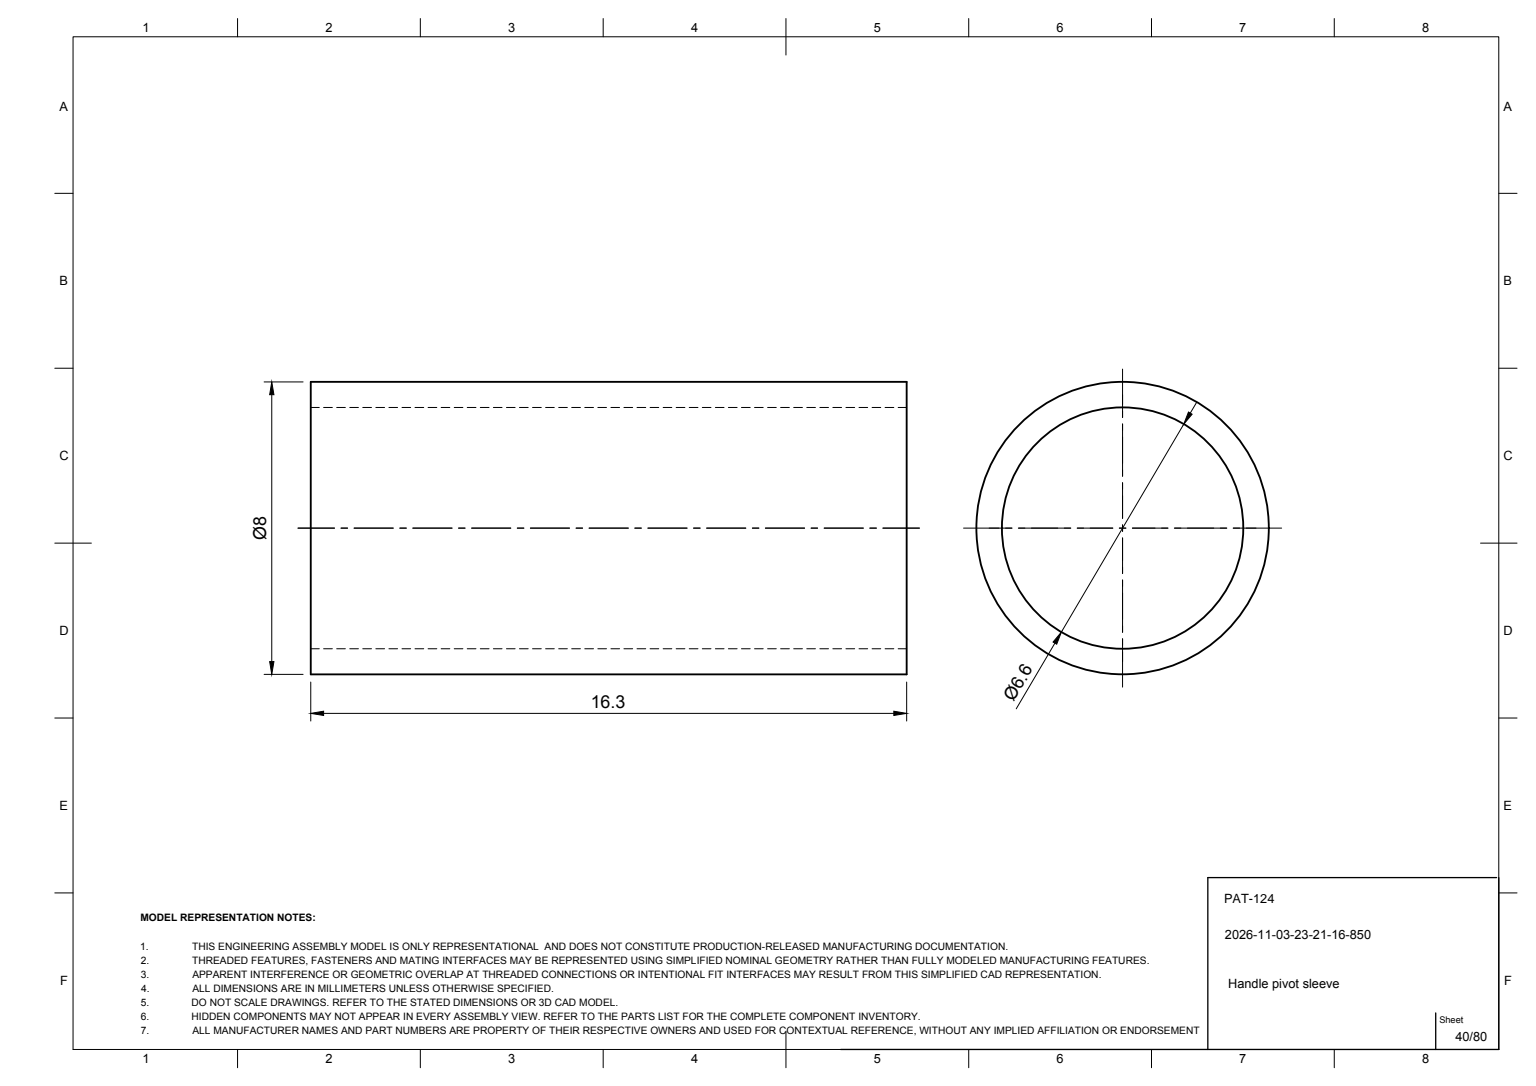
ISO-10303-21;
HEADER;
/* Generated by software containing ST-Developer
 * from STEP Tools, Inc. (www.steptools.com) 
 */

FILE_DESCRIPTION(
/* description */ ('XY cross-slide table'),
/* implementation_level */ '2;1');

FILE_NAME(
/* name */ 'Handle pivot sleeve.step',
/* time_stamp */ '2026-10-28T03:22:46-07:00',
/* author */ (''),
/* organization */ (''),
/* preprocessor_version */ 'ST-DEVELOPER v20.2',
/* originating_system */ 'Autodesk Translation Framework v15.17.0.0',
/* authorisation */ '');

FILE_SCHEMA (('AUTOMOTIVE_DESIGN { 1 0 10303 214 3 1 1 }'));
ENDSEC;

DATA;
#10=MECHANICAL_DESIGN_GEOMETRIC_PRESENTATION_REPRESENTATION('',(#1721),#62984);
#1540=SHAPE_REPRESENTATION_RELATIONSHIP('SRR','None',#63393,#1623);
#1623=ADVANCED_BREP_SHAPE_REPRESENTATION('',(#1831),#62930);
#1721=STYLED_ITEM('',(#63905),#1831);
#1831=MANIFOLD_SOLID_BREP('Body1',#23018);
#2077=FACE_BOUND('',#4968,.T.);
#2078=FACE_BOUND('',#4970,.T.);
#2541=PLANE('',#25079);
#2542=PLANE('',#25080);
#3461=FACE_OUTER_BOUND('',#4965,.T.);
#3462=FACE_OUTER_BOUND('',#4966,.T.);
#3463=FACE_OUTER_BOUND('',#4967,.T.);
#3464=FACE_OUTER_BOUND('',#4969,.T.);
#4965=EDGE_LOOP('',(#17732,#17733,#17734,#17735));
#4966=EDGE_LOOP('',(#17736,#17737,#17738,#17739));
#4967=EDGE_LOOP('',(#17740));
#4968=EDGE_LOOP('',(#17741));
#4969=EDGE_LOOP('',(#17742));
#4970=EDGE_LOOP('',(#17743));
#6569=LINE('',#47517,#8056);
#6570=LINE('',#47523,#8057);
#8056=VECTOR('',#29274,0.33);
#8057=VECTOR('',#29281,0.4);
#9287=CIRCLE('',#25074,0.33);
#9288=CIRCLE('',#25075,0.33);
#9289=CIRCLE('',#25077,0.4);
#9290=CIRCLE('',#25078,0.4);
#10727=VERTEX_POINT('',#47514);
#10728=VERTEX_POINT('',#47516);
#10729=VERTEX_POINT('',#47520);
#10730=VERTEX_POINT('',#47522);
#13250=EDGE_CURVE('',#10727,#10727,#9287,.T.);
#13251=EDGE_CURVE('',#10727,#10728,#6569,.T.);
#13252=EDGE_CURVE('',#10728,#10728,#9288,.T.);
#13253=EDGE_CURVE('',#10729,#10729,#9289,.T.);
#13254=EDGE_CURVE('',#10729,#10730,#6570,.T.);
#13255=EDGE_CURVE('',#10730,#10730,#9290,.T.);
#17732=ORIENTED_EDGE('',*,*,#13250,.F.);
#17733=ORIENTED_EDGE('',*,*,#13251,.T.);
#17734=ORIENTED_EDGE('',*,*,#13252,.T.);
#17735=ORIENTED_EDGE('',*,*,#13251,.F.);
#17736=ORIENTED_EDGE('',*,*,#13253,.F.);
#17737=ORIENTED_EDGE('',*,*,#13254,.T.);
#17738=ORIENTED_EDGE('',*,*,#13255,.T.);
#17739=ORIENTED_EDGE('',*,*,#13254,.F.);
#17740=ORIENTED_EDGE('',*,*,#13253,.T.);
#17741=ORIENTED_EDGE('',*,*,#13250,.T.);
#17742=ORIENTED_EDGE('',*,*,#13255,.F.);
#17743=ORIENTED_EDGE('',*,*,#13252,.F.);
#21329=CYLINDRICAL_SURFACE('',#25073,0.33);
#21330=CYLINDRICAL_SURFACE('',#25076,0.4);
#22242=ADVANCED_FACE('',(#3461),#21329,.F.);
#22243=ADVANCED_FACE('',(#3462),#21330,.T.);
#22244=ADVANCED_FACE('',(#3463,#2077),#2541,.T.);
#22245=ADVANCED_FACE('',(#3464,#2078),#2542,.F.);
#23018=CLOSED_SHELL('',(#22242,#22243,#22244,#22245));
#25072=AXIS2_PLACEMENT_3D('',#47512,#29268,#29269);
#25073=AXIS2_PLACEMENT_3D('',#47513,#29270,#29271);
#25074=AXIS2_PLACEMENT_3D('',#47515,#29272,#29273);
#25075=AXIS2_PLACEMENT_3D('',#47518,#29275,#29276);
#25076=AXIS2_PLACEMENT_3D('',#47519,#29277,#29278);
#25077=AXIS2_PLACEMENT_3D('',#47521,#29279,#29280);
#25078=AXIS2_PLACEMENT_3D('',#47524,#29282,#29283);
#25079=AXIS2_PLACEMENT_3D('',#47525,#29284,#29285);
#25080=AXIS2_PLACEMENT_3D('',#47526,#29286,#29287);
#29268=DIRECTION('axis',(0.,0.,1.));
#29269=DIRECTION('refdir',(1.,0.,0.));
#29270=DIRECTION('center_axis',(1.,0.,0.));
#29271=DIRECTION('ref_axis',(0.,0.,-1.));
#29272=DIRECTION('center_axis',(-1.,0.,0.));
#29273=DIRECTION('ref_axis',(0.,0.,-1.));
#29274=DIRECTION('',(-1.,0.,0.));
#29275=DIRECTION('center_axis',(-1.,0.,0.));
#29276=DIRECTION('ref_axis',(0.,0.,-1.));
#29277=DIRECTION('center_axis',(1.,0.,0.));
#29278=DIRECTION('ref_axis',(0.,0.,-1.));
#29279=DIRECTION('center_axis',(1.,0.,0.));
#29280=DIRECTION('ref_axis',(0.,0.,-1.));
#29281=DIRECTION('',(-1.,0.,0.));
#29282=DIRECTION('center_axis',(1.,0.,0.));
#29283=DIRECTION('ref_axis',(0.,0.,-1.));
#29284=DIRECTION('center_axis',(1.,0.,0.));
#29285=DIRECTION('ref_axis',(0.,0.,-1.));
#29286=DIRECTION('center_axis',(1.,0.,0.));
#29287=DIRECTION('ref_axis',(0.,0.,-1.));
#47512=CARTESIAN_POINT('',(0.,0.,0.));
#47513=CARTESIAN_POINT('Origin',(29.4,0.,6.5));
#47514=CARTESIAN_POINT('',(31.03,-4.04133443718627E-17,6.83));
#47515=CARTESIAN_POINT('Origin',(31.03,0.,6.5));
#47516=CARTESIAN_POINT('',(29.4,-4.04133443718627E-17,6.83));
#47517=CARTESIAN_POINT('',(29.4,-4.04133443718627E-17,6.83));
#47518=CARTESIAN_POINT('Origin',(29.4,0.,6.5));
#47519=CARTESIAN_POINT('Origin',(29.4,0.,6.5));
#47520=CARTESIAN_POINT('',(31.03,-4.89858719658942E-17,6.9));
#47521=CARTESIAN_POINT('Origin',(31.03,0.,6.5));
#47522=CARTESIAN_POINT('',(29.4,-4.89858719658942E-17,6.9));
#47523=CARTESIAN_POINT('',(29.4,-4.89858719658942E-17,6.9));
#47524=CARTESIAN_POINT('Origin',(29.4,0.,6.5));
#47525=CARTESIAN_POINT('Origin',(31.03,0.,6.5));
#47526=CARTESIAN_POINT('Origin',(29.4,0.,6.5));
#62831=UNCERTAINTY_MEASURE_WITH_UNIT(LENGTH_MEASURE(0.001),#62985,
'DISTANCE_ACCURACY_VALUE',
'Maximum model space distance between geometric entities at asserted c
onnectivities');
#62885=UNCERTAINTY_MEASURE_WITH_UNIT(LENGTH_MEASURE(0.001),#62985,
'DISTANCE_ACCURACY_VALUE',
'Maximum model space distance between geometric entities at asserted c
onnectivities');
#62930=(
GEOMETRIC_REPRESENTATION_CONTEXT(3)
GLOBAL_UNCERTAINTY_ASSIGNED_CONTEXT((#62831))
GLOBAL_UNIT_ASSIGNED_CONTEXT((#62985,#62987,#62988))
REPRESENTATION_CONTEXT('','3D')
);
#62984=(
GEOMETRIC_REPRESENTATION_CONTEXT(3)
GLOBAL_UNCERTAINTY_ASSIGNED_CONTEXT((#62885))
GLOBAL_UNIT_ASSIGNED_CONTEXT((#62985,#62987,#62988))
REPRESENTATION_CONTEXT('','3D')
);
#62985=(
LENGTH_UNIT()
NAMED_UNIT(*)
SI_UNIT(.CENTI.,.METRE.)
);
#62987=(
NAMED_UNIT(*)
PLANE_ANGLE_UNIT()
SI_UNIT($,.RADIAN.)
);
#62988=(
NAMED_UNIT(*)
SI_UNIT($,.STERADIAN.)
SOLID_ANGLE_UNIT()
);
#63033=SHAPE_DEFINITION_REPRESENTATION(#63164,#63393);
#63164=PRODUCT_DEFINITION_SHAPE('',$,#63492);
#63393=SHAPE_REPRESENTATION('',(#25072),#62930);
#63447=PRODUCT_DEFINITION_CONTEXT('part definition',#63743,'design');
#63492=PRODUCT_DEFINITION('Handle pivot sleeve','Handle pivot sleeve',#63590,
#63447);
#63590=PRODUCT_DEFINITION_FORMATION('',$,#63789);
#63743=APPLICATION_CONTEXT(
'Core Data for Automotive Mechanical Design Process');
#63744=PRODUCT_CONTEXT('part definition',#63743,'mechanical');
#63789=PRODUCT('Handle pivot sleeve','Handle pivot sleeve',
'Handle pivot sleeve',(#63744));
#63899=COLOUR_RGB('Sky Blue',0.24,0.69,0.87);
#63900=FILL_AREA_STYLE_COLOUR('',#63899);
#63901=FILL_AREA_STYLE('',(#63900));
#63902=SURFACE_STYLE_FILL_AREA(#63901);
#63903=SURFACE_SIDE_STYLE('',(#63902));
#63904=SURFACE_STYLE_USAGE(.BOTH.,#63903);
#63905=PRESENTATION_STYLE_ASSIGNMENT((#63904));
ENDSEC;
END-ISO-10303-21;
